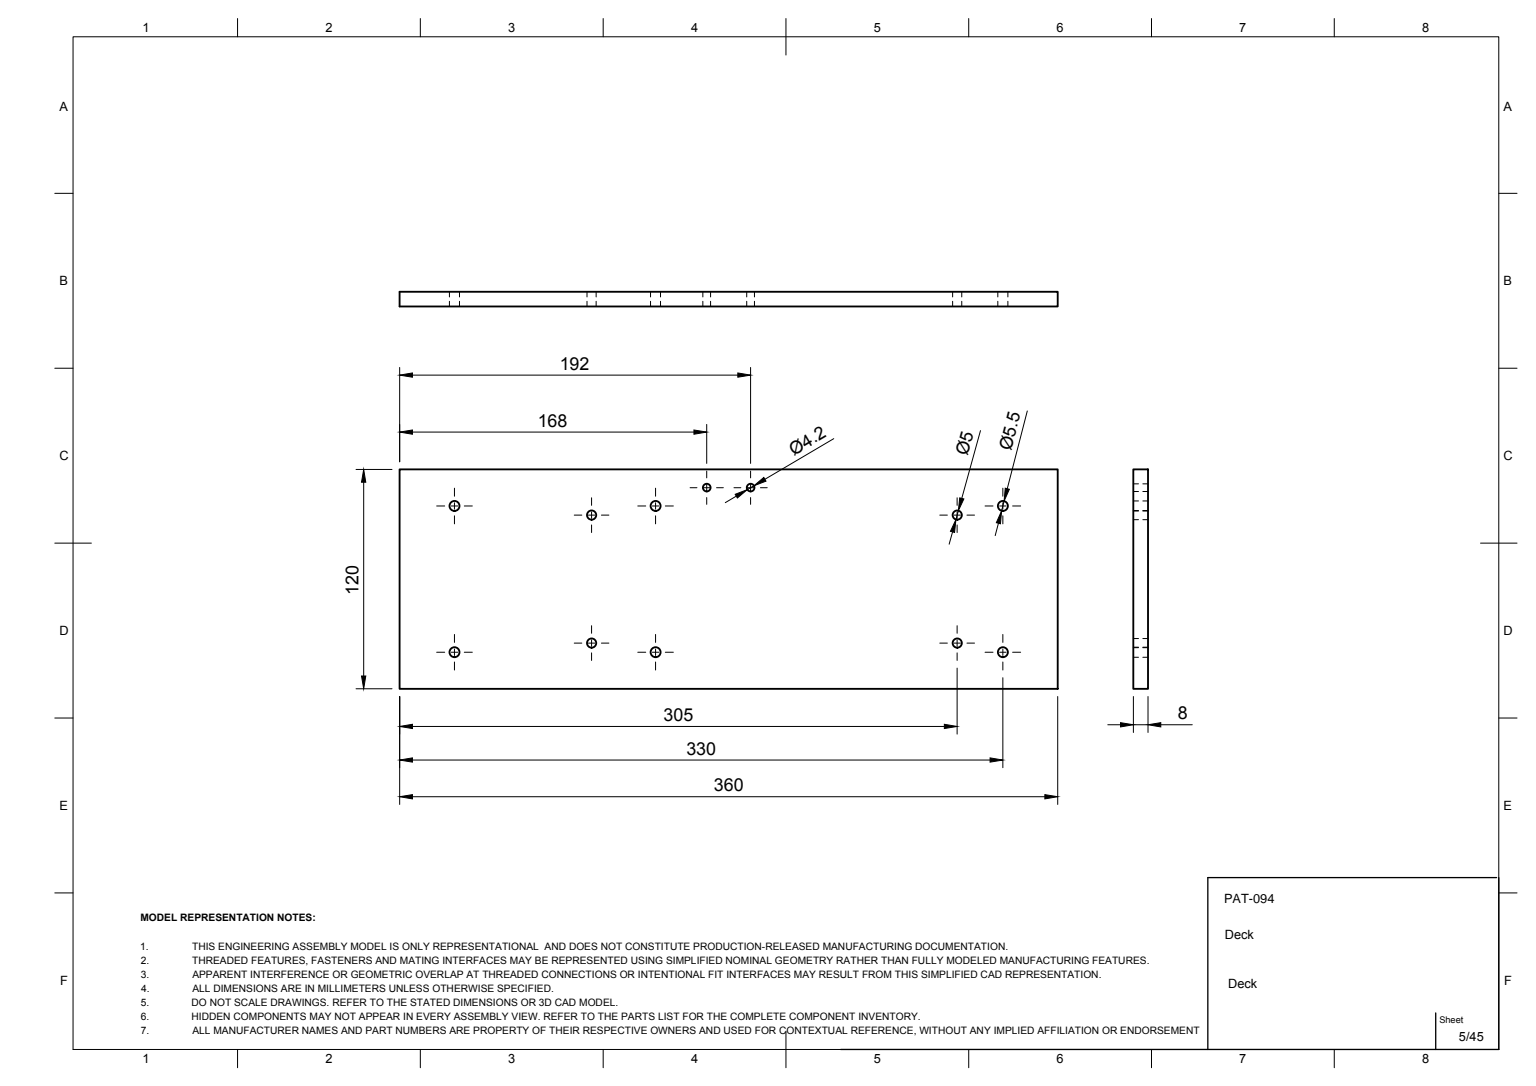
ISO-10303-21;
HEADER;
/* Generated by software containing ST-Developer
 * from STEP Tools, Inc. (www.steptools.com) 
 */

FILE_DESCRIPTION(
/* description */ ('Shaft runout checking stand'),
/* implementation_level */ '2;1');

FILE_NAME(
/* name */ 'Deck.step',
/* time_stamp */ '2026-11-02T21:12:33-08:00',
/* author */ (''),
/* organization */ (''),
/* preprocessor_version */ 'ST-DEVELOPER v20.2',
/* originating_system */ 'Autodesk Translation Framework v15.17.0.0',
/* authorisation */ '');

FILE_SCHEMA (('AUTOMOTIVE_DESIGN { 1 0 10303 214 3 1 1 }'));
ENDSEC;

DATA;
#10=MECHANICAL_DESIGN_GEOMETRIC_PRESENTATION_REPRESENTATION('',(#464),#11748);
#378=SHAPE_REPRESENTATION_RELATIONSHIP('SRR','None',#11927,#421);
#421=ADVANCED_BREP_SHAPE_REPRESENTATION('',(#515),#11703);
#464=STYLED_ITEM('',(#12169),#515);
#515=MANIFOLD_SOLID_BREP('Body1',#6207);
#564=FACE_BOUND('',#1472,.T.);
#565=FACE_BOUND('',#1473,.T.);
#566=FACE_BOUND('',#1474,.T.);
#567=FACE_BOUND('',#1475,.T.);
#568=FACE_BOUND('',#1476,.T.);
#569=FACE_BOUND('',#1477,.T.);
#570=FACE_BOUND('',#1478,.T.);
#571=FACE_BOUND('',#1479,.T.);
#572=FACE_BOUND('',#1480,.T.);
#573=FACE_BOUND('',#1481,.T.);
#574=FACE_BOUND('',#1482,.T.);
#575=FACE_BOUND('',#1483,.T.);
#576=FACE_BOUND('',#1485,.T.);
#577=FACE_BOUND('',#1486,.T.);
#578=FACE_BOUND('',#1487,.T.);
#579=FACE_BOUND('',#1488,.T.);
#580=FACE_BOUND('',#1489,.T.);
#581=FACE_BOUND('',#1490,.T.);
#582=FACE_BOUND('',#1491,.T.);
#583=FACE_BOUND('',#1492,.T.);
#584=FACE_BOUND('',#1493,.T.);
#585=FACE_BOUND('',#1494,.T.);
#586=FACE_BOUND('',#1495,.T.);
#587=FACE_BOUND('',#1496,.T.);
#675=CIRCLE('',#6788,0.21);
#676=CIRCLE('',#6789,0.21);
#677=CIRCLE('',#6791,0.21);
#678=CIRCLE('',#6792,0.21);
#679=CIRCLE('',#6794,0.25);
#680=CIRCLE('',#6795,0.25);
#681=CIRCLE('',#6797,0.25);
#682=CIRCLE('',#6798,0.25);
#683=CIRCLE('',#6800,0.25);
#684=CIRCLE('',#6801,0.25);
#685=CIRCLE('',#6803,0.25);
#686=CIRCLE('',#6804,0.25);
#687=CIRCLE('',#6806,0.275);
#688=CIRCLE('',#6807,0.275);
#689=CIRCLE('',#6809,0.275);
#690=CIRCLE('',#6810,0.275);
#691=CIRCLE('',#6812,0.275);
#692=CIRCLE('',#6813,0.275);
#693=CIRCLE('',#6815,0.275);
#694=CIRCLE('',#6816,0.275);
#695=CIRCLE('',#6818,0.275);
#696=CIRCLE('',#6819,0.275);
#697=CIRCLE('',#6821,0.275);
#698=CIRCLE('',#6822,0.275);
#939=CYLINDRICAL_SURFACE('',#6787,0.21);
#940=CYLINDRICAL_SURFACE('',#6790,0.21);
#941=CYLINDRICAL_SURFACE('',#6793,0.25);
#942=CYLINDRICAL_SURFACE('',#6796,0.25);
#943=CYLINDRICAL_SURFACE('',#6799,0.25);
#944=CYLINDRICAL_SURFACE('',#6802,0.25);
#945=CYLINDRICAL_SURFACE('',#6805,0.275);
#946=CYLINDRICAL_SURFACE('',#6808,0.275);
#947=CYLINDRICAL_SURFACE('',#6811,0.275);
#948=CYLINDRICAL_SURFACE('',#6814,0.275);
#949=CYLINDRICAL_SURFACE('',#6817,0.275);
#950=CYLINDRICAL_SURFACE('',#6820,0.275);
#1085=FACE_OUTER_BOUND('',#1455,.T.);
#1086=FACE_OUTER_BOUND('',#1456,.T.);
#1087=FACE_OUTER_BOUND('',#1457,.T.);
#1088=FACE_OUTER_BOUND('',#1458,.T.);
#1089=FACE_OUTER_BOUND('',#1459,.T.);
#1090=FACE_OUTER_BOUND('',#1460,.T.);
#1091=FACE_OUTER_BOUND('',#1461,.T.);
#1092=FACE_OUTER_BOUND('',#1462,.T.);
#1093=FACE_OUTER_BOUND('',#1463,.T.);
#1094=FACE_OUTER_BOUND('',#1464,.T.);
#1095=FACE_OUTER_BOUND('',#1465,.T.);
#1096=FACE_OUTER_BOUND('',#1466,.T.);
#1097=FACE_OUTER_BOUND('',#1467,.T.);
#1098=FACE_OUTER_BOUND('',#1468,.T.);
#1099=FACE_OUTER_BOUND('',#1469,.T.);
#1100=FACE_OUTER_BOUND('',#1470,.T.);
#1101=FACE_OUTER_BOUND('',#1471,.T.);
#1102=FACE_OUTER_BOUND('',#1484,.T.);
#1455=EDGE_LOOP('',(#4358,#4359,#4360,#4361));
#1456=EDGE_LOOP('',(#4362,#4363,#4364,#4365));
#1457=EDGE_LOOP('',(#4366,#4367,#4368,#4369));
#1458=EDGE_LOOP('',(#4370,#4371,#4372,#4373));
#1459=EDGE_LOOP('',(#4374,#4375,#4376,#4377));
#1460=EDGE_LOOP('',(#4378,#4379,#4380,#4381));
#1461=EDGE_LOOP('',(#4382,#4383,#4384,#4385));
#1462=EDGE_LOOP('',(#4386,#4387,#4388,#4389));
#1463=EDGE_LOOP('',(#4390,#4391,#4392,#4393));
#1464=EDGE_LOOP('',(#4394,#4395,#4396,#4397));
#1465=EDGE_LOOP('',(#4398,#4399,#4400,#4401));
#1466=EDGE_LOOP('',(#4402,#4403,#4404,#4405));
#1467=EDGE_LOOP('',(#4406,#4407,#4408,#4409));
#1468=EDGE_LOOP('',(#4410,#4411,#4412,#4413));
#1469=EDGE_LOOP('',(#4414,#4415,#4416,#4417));
#1470=EDGE_LOOP('',(#4418,#4419,#4420,#4421));
#1471=EDGE_LOOP('',(#4422,#4423,#4424,#4425));
#1472=EDGE_LOOP('',(#4426));
#1473=EDGE_LOOP('',(#4427));
#1474=EDGE_LOOP('',(#4428));
#1475=EDGE_LOOP('',(#4429));
#1476=EDGE_LOOP('',(#4430));
#1477=EDGE_LOOP('',(#4431));
#1478=EDGE_LOOP('',(#4432));
#1479=EDGE_LOOP('',(#4433));
#1480=EDGE_LOOP('',(#4434));
#1481=EDGE_LOOP('',(#4435));
#1482=EDGE_LOOP('',(#4436));
#1483=EDGE_LOOP('',(#4437));
#1484=EDGE_LOOP('',(#4438,#4439,#4440,#4441));
#1485=EDGE_LOOP('',(#4442));
#1486=EDGE_LOOP('',(#4443));
#1487=EDGE_LOOP('',(#4444));
#1488=EDGE_LOOP('',(#4445));
#1489=EDGE_LOOP('',(#4446));
#1490=EDGE_LOOP('',(#4447));
#1491=EDGE_LOOP('',(#4448));
#1492=EDGE_LOOP('',(#4449));
#1493=EDGE_LOOP('',(#4450));
#1494=EDGE_LOOP('',(#4451));
#1495=EDGE_LOOP('',(#4452));
#1496=EDGE_LOOP('',(#4453));
#2018=LINE('',#9755,#2485);
#2019=LINE('',#9761,#2486);
#2020=LINE('',#9767,#2487);
#2021=LINE('',#9773,#2488);
#2022=LINE('',#9779,#2489);
#2023=LINE('',#9785,#2490);
#2024=LINE('',#9791,#2491);
#2025=LINE('',#9797,#2492);
#2026=LINE('',#9803,#2493);
#2027=LINE('',#9809,#2494);
#2028=LINE('',#9815,#2495);
#2029=LINE('',#9821,#2496);
#2030=LINE('',#9826,#2497);
#2031=LINE('',#9828,#2498);
#2032=LINE('',#9830,#2499);
#2033=LINE('',#9831,#2500);
#2034=LINE('',#9834,#2501);
#2035=LINE('',#9836,#2502);
#2036=LINE('',#9837,#2503);
#2037=LINE('',#9840,#2504);
#2038=LINE('',#9842,#2505);
#2039=LINE('',#9843,#2506);
#2040=LINE('',#9845,#2507);
#2041=LINE('',#9846,#2508);
#2485=VECTOR('',#7735,0.21);
#2486=VECTOR('',#7742,0.21);
#2487=VECTOR('',#7749,0.25);
#2488=VECTOR('',#7756,0.25);
#2489=VECTOR('',#7763,0.25);
#2490=VECTOR('',#7770,0.25);
#2491=VECTOR('',#7777,0.275);
#2492=VECTOR('',#7784,0.275);
#2493=VECTOR('',#7791,0.275);
#2494=VECTOR('',#7798,0.275);
#2495=VECTOR('',#7805,0.275);
#2496=VECTOR('',#7812,0.275);
#2497=VECTOR('',#7817,1.);
#2498=VECTOR('',#7818,1.);
#2499=VECTOR('',#7819,1.);
#2500=VECTOR('',#7820,1.);
#2501=VECTOR('',#7823,1.);
#2502=VECTOR('',#7824,1.);
#2503=VECTOR('',#7825,1.);
#2504=VECTOR('',#7828,1.);
#2505=VECTOR('',#7829,1.);
#2506=VECTOR('',#7830,1.);
#2507=VECTOR('',#7833,1.);
#2508=VECTOR('',#7834,1.);
#2909=VERTEX_POINT('',#9752);
#2910=VERTEX_POINT('',#9754);
#2911=VERTEX_POINT('',#9758);
#2912=VERTEX_POINT('',#9760);
#2913=VERTEX_POINT('',#9764);
#2914=VERTEX_POINT('',#9766);
#2915=VERTEX_POINT('',#9770);
#2916=VERTEX_POINT('',#9772);
#2917=VERTEX_POINT('',#9776);
#2918=VERTEX_POINT('',#9778);
#2919=VERTEX_POINT('',#9782);
#2920=VERTEX_POINT('',#9784);
#2921=VERTEX_POINT('',#9788);
#2922=VERTEX_POINT('',#9790);
#2923=VERTEX_POINT('',#9794);
#2924=VERTEX_POINT('',#9796);
#2925=VERTEX_POINT('',#9800);
#2926=VERTEX_POINT('',#9802);
#2927=VERTEX_POINT('',#9806);
#2928=VERTEX_POINT('',#9808);
#2929=VERTEX_POINT('',#9812);
#2930=VERTEX_POINT('',#9814);
#2931=VERTEX_POINT('',#9818);
#2932=VERTEX_POINT('',#9820);
#2933=VERTEX_POINT('',#9824);
#2934=VERTEX_POINT('',#9825);
#2935=VERTEX_POINT('',#9827);
#2936=VERTEX_POINT('',#9829);
#2937=VERTEX_POINT('',#9833);
#2938=VERTEX_POINT('',#9835);
#2939=VERTEX_POINT('',#9839);
#2940=VERTEX_POINT('',#9841);
#3465=EDGE_CURVE('',#2909,#2909,#675,.T.);
#3466=EDGE_CURVE('',#2909,#2910,#2018,.T.);
#3467=EDGE_CURVE('',#2910,#2910,#676,.T.);
#3468=EDGE_CURVE('',#2911,#2911,#677,.T.);
#3469=EDGE_CURVE('',#2911,#2912,#2019,.T.);
#3470=EDGE_CURVE('',#2912,#2912,#678,.T.);
#3471=EDGE_CURVE('',#2913,#2913,#679,.T.);
#3472=EDGE_CURVE('',#2913,#2914,#2020,.T.);
#3473=EDGE_CURVE('',#2914,#2914,#680,.T.);
#3474=EDGE_CURVE('',#2915,#2915,#681,.T.);
#3475=EDGE_CURVE('',#2915,#2916,#2021,.T.);
#3476=EDGE_CURVE('',#2916,#2916,#682,.T.);
#3477=EDGE_CURVE('',#2917,#2917,#683,.T.);
#3478=EDGE_CURVE('',#2917,#2918,#2022,.T.);
#3479=EDGE_CURVE('',#2918,#2918,#684,.T.);
#3480=EDGE_CURVE('',#2919,#2919,#685,.T.);
#3481=EDGE_CURVE('',#2919,#2920,#2023,.T.);
#3482=EDGE_CURVE('',#2920,#2920,#686,.T.);
#3483=EDGE_CURVE('',#2921,#2921,#687,.T.);
#3484=EDGE_CURVE('',#2921,#2922,#2024,.T.);
#3485=EDGE_CURVE('',#2922,#2922,#688,.T.);
#3486=EDGE_CURVE('',#2923,#2923,#689,.T.);
#3487=EDGE_CURVE('',#2923,#2924,#2025,.T.);
#3488=EDGE_CURVE('',#2924,#2924,#690,.T.);
#3489=EDGE_CURVE('',#2925,#2925,#691,.T.);
#3490=EDGE_CURVE('',#2925,#2926,#2026,.T.);
#3491=EDGE_CURVE('',#2926,#2926,#692,.T.);
#3492=EDGE_CURVE('',#2927,#2927,#693,.T.);
#3493=EDGE_CURVE('',#2927,#2928,#2027,.T.);
#3494=EDGE_CURVE('',#2928,#2928,#694,.T.);
#3495=EDGE_CURVE('',#2929,#2929,#695,.T.);
#3496=EDGE_CURVE('',#2929,#2930,#2028,.T.);
#3497=EDGE_CURVE('',#2930,#2930,#696,.T.);
#3498=EDGE_CURVE('',#2931,#2931,#697,.T.);
#3499=EDGE_CURVE('',#2931,#2932,#2029,.T.);
#3500=EDGE_CURVE('',#2932,#2932,#698,.T.);
#3501=EDGE_CURVE('',#2933,#2934,#2030,.T.);
#3502=EDGE_CURVE('',#2934,#2935,#2031,.T.);
#3503=EDGE_CURVE('',#2936,#2935,#2032,.T.);
#3504=EDGE_CURVE('',#2933,#2936,#2033,.T.);
#3505=EDGE_CURVE('',#2937,#2933,#2034,.T.);
#3506=EDGE_CURVE('',#2938,#2936,#2035,.T.);
#3507=EDGE_CURVE('',#2937,#2938,#2036,.T.);
#3508=EDGE_CURVE('',#2939,#2937,#2037,.T.);
#3509=EDGE_CURVE('',#2940,#2938,#2038,.T.);
#3510=EDGE_CURVE('',#2939,#2940,#2039,.T.);
#3511=EDGE_CURVE('',#2934,#2939,#2040,.T.);
#3512=EDGE_CURVE('',#2935,#2940,#2041,.T.);
#4358=ORIENTED_EDGE('',*,*,#3465,.F.);
#4359=ORIENTED_EDGE('',*,*,#3466,.T.);
#4360=ORIENTED_EDGE('',*,*,#3467,.F.);
#4361=ORIENTED_EDGE('',*,*,#3466,.F.);
#4362=ORIENTED_EDGE('',*,*,#3468,.F.);
#4363=ORIENTED_EDGE('',*,*,#3469,.T.);
#4364=ORIENTED_EDGE('',*,*,#3470,.F.);
#4365=ORIENTED_EDGE('',*,*,#3469,.F.);
#4366=ORIENTED_EDGE('',*,*,#3471,.F.);
#4367=ORIENTED_EDGE('',*,*,#3472,.T.);
#4368=ORIENTED_EDGE('',*,*,#3473,.F.);
#4369=ORIENTED_EDGE('',*,*,#3472,.F.);
#4370=ORIENTED_EDGE('',*,*,#3474,.F.);
#4371=ORIENTED_EDGE('',*,*,#3475,.T.);
#4372=ORIENTED_EDGE('',*,*,#3476,.F.);
#4373=ORIENTED_EDGE('',*,*,#3475,.F.);
#4374=ORIENTED_EDGE('',*,*,#3477,.F.);
#4375=ORIENTED_EDGE('',*,*,#3478,.T.);
#4376=ORIENTED_EDGE('',*,*,#3479,.F.);
#4377=ORIENTED_EDGE('',*,*,#3478,.F.);
#4378=ORIENTED_EDGE('',*,*,#3480,.F.);
#4379=ORIENTED_EDGE('',*,*,#3481,.T.);
#4380=ORIENTED_EDGE('',*,*,#3482,.F.);
#4381=ORIENTED_EDGE('',*,*,#3481,.F.);
#4382=ORIENTED_EDGE('',*,*,#3483,.F.);
#4383=ORIENTED_EDGE('',*,*,#3484,.T.);
#4384=ORIENTED_EDGE('',*,*,#3485,.F.);
#4385=ORIENTED_EDGE('',*,*,#3484,.F.);
#4386=ORIENTED_EDGE('',*,*,#3486,.F.);
#4387=ORIENTED_EDGE('',*,*,#3487,.T.);
#4388=ORIENTED_EDGE('',*,*,#3488,.F.);
#4389=ORIENTED_EDGE('',*,*,#3487,.F.);
#4390=ORIENTED_EDGE('',*,*,#3489,.F.);
#4391=ORIENTED_EDGE('',*,*,#3490,.T.);
#4392=ORIENTED_EDGE('',*,*,#3491,.F.);
#4393=ORIENTED_EDGE('',*,*,#3490,.F.);
#4394=ORIENTED_EDGE('',*,*,#3492,.F.);
#4395=ORIENTED_EDGE('',*,*,#3493,.T.);
#4396=ORIENTED_EDGE('',*,*,#3494,.F.);
#4397=ORIENTED_EDGE('',*,*,#3493,.F.);
#4398=ORIENTED_EDGE('',*,*,#3495,.F.);
#4399=ORIENTED_EDGE('',*,*,#3496,.T.);
#4400=ORIENTED_EDGE('',*,*,#3497,.F.);
#4401=ORIENTED_EDGE('',*,*,#3496,.F.);
#4402=ORIENTED_EDGE('',*,*,#3498,.F.);
#4403=ORIENTED_EDGE('',*,*,#3499,.T.);
#4404=ORIENTED_EDGE('',*,*,#3500,.F.);
#4405=ORIENTED_EDGE('',*,*,#3499,.F.);
#4406=ORIENTED_EDGE('',*,*,#3501,.T.);
#4407=ORIENTED_EDGE('',*,*,#3502,.T.);
#4408=ORIENTED_EDGE('',*,*,#3503,.F.);
#4409=ORIENTED_EDGE('',*,*,#3504,.F.);
#4410=ORIENTED_EDGE('',*,*,#3505,.T.);
#4411=ORIENTED_EDGE('',*,*,#3504,.T.);
#4412=ORIENTED_EDGE('',*,*,#3506,.F.);
#4413=ORIENTED_EDGE('',*,*,#3507,.F.);
#4414=ORIENTED_EDGE('',*,*,#3508,.T.);
#4415=ORIENTED_EDGE('',*,*,#3507,.T.);
#4416=ORIENTED_EDGE('',*,*,#3509,.F.);
#4417=ORIENTED_EDGE('',*,*,#3510,.F.);
#4418=ORIENTED_EDGE('',*,*,#3511,.T.);
#4419=ORIENTED_EDGE('',*,*,#3510,.T.);
#4420=ORIENTED_EDGE('',*,*,#3512,.F.);
#4421=ORIENTED_EDGE('',*,*,#3502,.F.);
#4422=ORIENTED_EDGE('',*,*,#3512,.T.);
#4423=ORIENTED_EDGE('',*,*,#3509,.T.);
#4424=ORIENTED_EDGE('',*,*,#3506,.T.);
#4425=ORIENTED_EDGE('',*,*,#3503,.T.);
#4426=ORIENTED_EDGE('',*,*,#3473,.T.);
#4427=ORIENTED_EDGE('',*,*,#3476,.T.);
#4428=ORIENTED_EDGE('',*,*,#3485,.T.);
#4429=ORIENTED_EDGE('',*,*,#3488,.T.);
#4430=ORIENTED_EDGE('',*,*,#3491,.T.);
#4431=ORIENTED_EDGE('',*,*,#3494,.T.);
#4432=ORIENTED_EDGE('',*,*,#3497,.T.);
#4433=ORIENTED_EDGE('',*,*,#3500,.T.);
#4434=ORIENTED_EDGE('',*,*,#3482,.T.);
#4435=ORIENTED_EDGE('',*,*,#3479,.T.);
#4436=ORIENTED_EDGE('',*,*,#3470,.T.);
#4437=ORIENTED_EDGE('',*,*,#3467,.T.);
#4438=ORIENTED_EDGE('',*,*,#3511,.F.);
#4439=ORIENTED_EDGE('',*,*,#3501,.F.);
#4440=ORIENTED_EDGE('',*,*,#3505,.F.);
#4441=ORIENTED_EDGE('',*,*,#3508,.F.);
#4442=ORIENTED_EDGE('',*,*,#3471,.T.);
#4443=ORIENTED_EDGE('',*,*,#3474,.T.);
#4444=ORIENTED_EDGE('',*,*,#3483,.T.);
#4445=ORIENTED_EDGE('',*,*,#3486,.T.);
#4446=ORIENTED_EDGE('',*,*,#3489,.T.);
#4447=ORIENTED_EDGE('',*,*,#3492,.T.);
#4448=ORIENTED_EDGE('',*,*,#3495,.T.);
#4449=ORIENTED_EDGE('',*,*,#3498,.T.);
#4450=ORIENTED_EDGE('',*,*,#3480,.T.);
#4451=ORIENTED_EDGE('',*,*,#3477,.T.);
#4452=ORIENTED_EDGE('',*,*,#3468,.T.);
#4453=ORIENTED_EDGE('',*,*,#3465,.T.);
#5650=PLANE('',#6823);
#5651=PLANE('',#6824);
#5652=PLANE('',#6825);
#5653=PLANE('',#6826);
#5654=PLANE('',#6827);
#5655=PLANE('',#6828);
#5885=ADVANCED_FACE('',(#1085),#939,.F.);
#5886=ADVANCED_FACE('',(#1086),#940,.F.);
#5887=ADVANCED_FACE('',(#1087),#941,.F.);
#5888=ADVANCED_FACE('',(#1088),#942,.F.);
#5889=ADVANCED_FACE('',(#1089),#943,.F.);
#5890=ADVANCED_FACE('',(#1090),#944,.F.);
#5891=ADVANCED_FACE('',(#1091),#945,.F.);
#5892=ADVANCED_FACE('',(#1092),#946,.F.);
#5893=ADVANCED_FACE('',(#1093),#947,.F.);
#5894=ADVANCED_FACE('',(#1094),#948,.F.);
#5895=ADVANCED_FACE('',(#1095),#949,.F.);
#5896=ADVANCED_FACE('',(#1096),#950,.F.);
#5897=ADVANCED_FACE('',(#1097),#5650,.T.);
#5898=ADVANCED_FACE('',(#1098),#5651,.T.);
#5899=ADVANCED_FACE('',(#1099),#5652,.T.);
#5900=ADVANCED_FACE('',(#1100),#5653,.T.);
#5901=ADVANCED_FACE('',(#1101,#564,#565,#566,#567,#568,#569,#570,#571,#572,
#573,#574,#575),#5654,.T.);
#5902=ADVANCED_FACE('',(#1102,#576,#577,#578,#579,#580,#581,#582,#583,#584,
#585,#586,#587),#5655,.F.);
#6207=CLOSED_SHELL('',(#5885,#5886,#5887,#5888,#5889,#5890,#5891,#5892,
#5893,#5894,#5895,#5896,#5897,#5898,#5899,#5900,#5901,#5902));
#6786=AXIS2_PLACEMENT_3D('',#9750,#7729,#7730);
#6787=AXIS2_PLACEMENT_3D('',#9751,#7731,#7732);
#6788=AXIS2_PLACEMENT_3D('',#9753,#7733,#7734);
#6789=AXIS2_PLACEMENT_3D('',#9756,#7736,#7737);
#6790=AXIS2_PLACEMENT_3D('',#9757,#7738,#7739);
#6791=AXIS2_PLACEMENT_3D('',#9759,#7740,#7741);
#6792=AXIS2_PLACEMENT_3D('',#9762,#7743,#7744);
#6793=AXIS2_PLACEMENT_3D('',#9763,#7745,#7746);
#6794=AXIS2_PLACEMENT_3D('',#9765,#7747,#7748);
#6795=AXIS2_PLACEMENT_3D('',#9768,#7750,#7751);
#6796=AXIS2_PLACEMENT_3D('',#9769,#7752,#7753);
#6797=AXIS2_PLACEMENT_3D('',#9771,#7754,#7755);
#6798=AXIS2_PLACEMENT_3D('',#9774,#7757,#7758);
#6799=AXIS2_PLACEMENT_3D('',#9775,#7759,#7760);
#6800=AXIS2_PLACEMENT_3D('',#9777,#7761,#7762);
#6801=AXIS2_PLACEMENT_3D('',#9780,#7764,#7765);
#6802=AXIS2_PLACEMENT_3D('',#9781,#7766,#7767);
#6803=AXIS2_PLACEMENT_3D('',#9783,#7768,#7769);
#6804=AXIS2_PLACEMENT_3D('',#9786,#7771,#7772);
#6805=AXIS2_PLACEMENT_3D('',#9787,#7773,#7774);
#6806=AXIS2_PLACEMENT_3D('',#9789,#7775,#7776);
#6807=AXIS2_PLACEMENT_3D('',#9792,#7778,#7779);
#6808=AXIS2_PLACEMENT_3D('',#9793,#7780,#7781);
#6809=AXIS2_PLACEMENT_3D('',#9795,#7782,#7783);
#6810=AXIS2_PLACEMENT_3D('',#9798,#7785,#7786);
#6811=AXIS2_PLACEMENT_3D('',#9799,#7787,#7788);
#6812=AXIS2_PLACEMENT_3D('',#9801,#7789,#7790);
#6813=AXIS2_PLACEMENT_3D('',#9804,#7792,#7793);
#6814=AXIS2_PLACEMENT_3D('',#9805,#7794,#7795);
#6815=AXIS2_PLACEMENT_3D('',#9807,#7796,#7797);
#6816=AXIS2_PLACEMENT_3D('',#9810,#7799,#7800);
#6817=AXIS2_PLACEMENT_3D('',#9811,#7801,#7802);
#6818=AXIS2_PLACEMENT_3D('',#9813,#7803,#7804);
#6819=AXIS2_PLACEMENT_3D('',#9816,#7806,#7807);
#6820=AXIS2_PLACEMENT_3D('',#9817,#7808,#7809);
#6821=AXIS2_PLACEMENT_3D('',#9819,#7810,#7811);
#6822=AXIS2_PLACEMENT_3D('',#9822,#7813,#7814);
#6823=AXIS2_PLACEMENT_3D('',#9823,#7815,#7816);
#6824=AXIS2_PLACEMENT_3D('',#9832,#7821,#7822);
#6825=AXIS2_PLACEMENT_3D('',#9838,#7826,#7827);
#6826=AXIS2_PLACEMENT_3D('',#9844,#7831,#7832);
#6827=AXIS2_PLACEMENT_3D('',#9847,#7835,#7836);
#6828=AXIS2_PLACEMENT_3D('',#9848,#7837,#7838);
#7729=DIRECTION('axis',(0.,0.,1.));
#7730=DIRECTION('refdir',(1.,0.,0.));
#7731=DIRECTION('center_axis',(0.,0.,1.));
#7732=DIRECTION('ref_axis',(1.,0.,0.));
#7733=DIRECTION('center_axis',(0.,0.,1.));
#7734=DIRECTION('ref_axis',(1.,0.,0.));
#7735=DIRECTION('',(0.,0.,1.));
#7736=DIRECTION('center_axis',(0.,0.,-1.));
#7737=DIRECTION('ref_axis',(1.,0.,0.));
#7738=DIRECTION('center_axis',(0.,0.,1.));
#7739=DIRECTION('ref_axis',(1.,0.,0.));
#7740=DIRECTION('center_axis',(0.,0.,1.));
#7741=DIRECTION('ref_axis',(1.,0.,0.));
#7742=DIRECTION('',(0.,0.,1.));
#7743=DIRECTION('center_axis',(0.,0.,-1.));
#7744=DIRECTION('ref_axis',(1.,0.,0.));
#7745=DIRECTION('center_axis',(0.,0.,1.));
#7746=DIRECTION('ref_axis',(1.,0.,0.));
#7747=DIRECTION('center_axis',(0.,0.,1.));
#7748=DIRECTION('ref_axis',(1.,0.,0.));
#7749=DIRECTION('',(0.,0.,1.));
#7750=DIRECTION('center_axis',(0.,0.,-1.));
#7751=DIRECTION('ref_axis',(1.,0.,0.));
#7752=DIRECTION('center_axis',(0.,0.,1.));
#7753=DIRECTION('ref_axis',(1.,0.,0.));
#7754=DIRECTION('center_axis',(0.,0.,1.));
#7755=DIRECTION('ref_axis',(1.,0.,0.));
#7756=DIRECTION('',(0.,0.,1.));
#7757=DIRECTION('center_axis',(0.,0.,-1.));
#7758=DIRECTION('ref_axis',(1.,0.,0.));
#7759=DIRECTION('center_axis',(0.,0.,1.));
#7760=DIRECTION('ref_axis',(1.,0.,0.));
#7761=DIRECTION('center_axis',(0.,0.,1.));
#7762=DIRECTION('ref_axis',(1.,0.,0.));
#7763=DIRECTION('',(0.,0.,1.));
#7764=DIRECTION('center_axis',(0.,0.,-1.));
#7765=DIRECTION('ref_axis',(1.,0.,0.));
#7766=DIRECTION('center_axis',(0.,0.,1.));
#7767=DIRECTION('ref_axis',(1.,0.,0.));
#7768=DIRECTION('center_axis',(0.,0.,1.));
#7769=DIRECTION('ref_axis',(1.,0.,0.));
#7770=DIRECTION('',(0.,0.,1.));
#7771=DIRECTION('center_axis',(0.,0.,-1.));
#7772=DIRECTION('ref_axis',(1.,0.,0.));
#7773=DIRECTION('center_axis',(0.,0.,1.));
#7774=DIRECTION('ref_axis',(1.,0.,0.));
#7775=DIRECTION('center_axis',(0.,0.,1.));
#7776=DIRECTION('ref_axis',(1.,0.,0.));
#7777=DIRECTION('',(0.,0.,1.));
#7778=DIRECTION('center_axis',(0.,0.,-1.));
#7779=DIRECTION('ref_axis',(1.,0.,0.));
#7780=DIRECTION('center_axis',(0.,0.,1.));
#7781=DIRECTION('ref_axis',(1.,0.,0.));
#7782=DIRECTION('center_axis',(0.,0.,1.));
#7783=DIRECTION('ref_axis',(1.,0.,0.));
#7784=DIRECTION('',(0.,0.,1.));
#7785=DIRECTION('center_axis',(0.,0.,-1.));
#7786=DIRECTION('ref_axis',(1.,0.,0.));
#7787=DIRECTION('center_axis',(0.,0.,1.));
#7788=DIRECTION('ref_axis',(1.,0.,0.));
#7789=DIRECTION('center_axis',(0.,0.,1.));
#7790=DIRECTION('ref_axis',(1.,0.,0.));
#7791=DIRECTION('',(0.,0.,1.));
#7792=DIRECTION('center_axis',(0.,0.,-1.));
#7793=DIRECTION('ref_axis',(1.,0.,0.));
#7794=DIRECTION('center_axis',(0.,0.,1.));
#7795=DIRECTION('ref_axis',(1.,0.,0.));
#7796=DIRECTION('center_axis',(0.,0.,1.));
#7797=DIRECTION('ref_axis',(1.,0.,0.));
#7798=DIRECTION('',(0.,0.,1.));
#7799=DIRECTION('center_axis',(0.,0.,-1.));
#7800=DIRECTION('ref_axis',(1.,0.,0.));
#7801=DIRECTION('center_axis',(0.,0.,1.));
#7802=DIRECTION('ref_axis',(1.,0.,0.));
#7803=DIRECTION('center_axis',(0.,0.,1.));
#7804=DIRECTION('ref_axis',(1.,0.,0.));
#7805=DIRECTION('',(0.,0.,1.));
#7806=DIRECTION('center_axis',(0.,0.,-1.));
#7807=DIRECTION('ref_axis',(1.,0.,0.));
#7808=DIRECTION('center_axis',(0.,0.,1.));
#7809=DIRECTION('ref_axis',(1.,0.,0.));
#7810=DIRECTION('center_axis',(0.,0.,1.));
#7811=DIRECTION('ref_axis',(1.,0.,0.));
#7812=DIRECTION('',(0.,0.,1.));
#7813=DIRECTION('center_axis',(0.,0.,-1.));
#7814=DIRECTION('ref_axis',(1.,0.,0.));
#7815=DIRECTION('center_axis',(0.,1.,0.));
#7816=DIRECTION('ref_axis',(-1.,0.,0.));
#7817=DIRECTION('',(-1.,0.,0.));
#7818=DIRECTION('',(0.,0.,1.));
#7819=DIRECTION('',(-1.,0.,0.));
#7820=DIRECTION('',(0.,0.,1.));
#7821=DIRECTION('center_axis',(1.,0.,0.));
#7822=DIRECTION('ref_axis',(0.,1.,0.));
#7823=DIRECTION('',(0.,1.,0.));
#7824=DIRECTION('',(0.,1.,0.));
#7825=DIRECTION('',(0.,0.,1.));
#7826=DIRECTION('center_axis',(0.,-1.,0.));
#7827=DIRECTION('ref_axis',(1.,0.,0.));
#7828=DIRECTION('',(1.,0.,0.));
#7829=DIRECTION('',(1.,0.,0.));
#7830=DIRECTION('',(0.,0.,1.));
#7831=DIRECTION('center_axis',(-1.,0.,0.));
#7832=DIRECTION('ref_axis',(0.,-1.,0.));
#7833=DIRECTION('',(0.,-1.,0.));
#7834=DIRECTION('',(0.,-1.,0.));
#7835=DIRECTION('center_axis',(0.,0.,1.));
#7836=DIRECTION('ref_axis',(1.,0.,0.));
#7837=DIRECTION('center_axis',(0.,0.,1.));
#7838=DIRECTION('ref_axis',(1.,0.,0.));
#9750=CARTESIAN_POINT('',(0.,0.,0.));
#9751=CARTESIAN_POINT('Origin',(5.,-1.2,1.9));
#9752=CARTESIAN_POINT('',(4.79,-1.2,2.));
#9753=CARTESIAN_POINT('Origin',(5.,-1.2,2.));
#9754=CARTESIAN_POINT('',(4.79,-1.2,2.8));
#9755=CARTESIAN_POINT('',(4.79,-1.2,1.9));
#9756=CARTESIAN_POINT('Origin',(5.,-1.2,2.8));
#9757=CARTESIAN_POINT('Origin',(5.,1.2,1.9));
#9758=CARTESIAN_POINT('',(4.79,1.2,2.));
#9759=CARTESIAN_POINT('Origin',(5.,1.2,2.));
#9760=CARTESIAN_POINT('',(4.79,1.2,2.8));
#9761=CARTESIAN_POINT('',(4.79,1.2,1.9));
#9762=CARTESIAN_POINT('Origin',(5.,1.2,2.8));
#9763=CARTESIAN_POINT('Origin',(-3.5,7.5,1.9));
#9764=CARTESIAN_POINT('',(-3.75,7.5,2.));
#9765=CARTESIAN_POINT('Origin',(-3.5,7.5,2.));
#9766=CARTESIAN_POINT('',(-3.75,7.5,2.8));
#9767=CARTESIAN_POINT('',(-3.75,7.5,1.9));
#9768=CARTESIAN_POINT('Origin',(-3.5,7.5,2.8));
#9769=CARTESIAN_POINT('Origin',(3.5,7.5,1.9));
#9770=CARTESIAN_POINT('',(3.25,7.5,2.));
#9771=CARTESIAN_POINT('Origin',(3.5,7.5,2.));
#9772=CARTESIAN_POINT('',(3.25,7.5,2.8));
#9773=CARTESIAN_POINT('',(3.25,7.5,1.9));
#9774=CARTESIAN_POINT('Origin',(3.5,7.5,2.8));
#9775=CARTESIAN_POINT('Origin',(-3.5,-12.5,1.9));
#9776=CARTESIAN_POINT('',(-3.75,-12.5,2.));
#9777=CARTESIAN_POINT('Origin',(-3.5,-12.5,2.));
#9778=CARTESIAN_POINT('',(-3.75,-12.5,2.8));
#9779=CARTESIAN_POINT('',(-3.75,-12.5,1.9));
#9780=CARTESIAN_POINT('Origin',(-3.5,-12.5,2.8));
#9781=CARTESIAN_POINT('Origin',(3.5,-12.5,1.9));
#9782=CARTESIAN_POINT('',(3.25,-12.5,2.));
#9783=CARTESIAN_POINT('Origin',(3.5,-12.5,2.));
#9784=CARTESIAN_POINT('',(3.25,-12.5,2.8));
#9785=CARTESIAN_POINT('',(3.25,-12.5,1.9));
#9786=CARTESIAN_POINT('Origin',(3.5,-12.5,2.8));
#9787=CARTESIAN_POINT('Origin',(4.,4.,1.9));
#9788=CARTESIAN_POINT('',(3.725,4.,2.));
#9789=CARTESIAN_POINT('Origin',(4.,4.,2.));
#9790=CARTESIAN_POINT('',(3.725,4.,2.8));
#9791=CARTESIAN_POINT('',(3.725,4.,1.9));
#9792=CARTESIAN_POINT('Origin',(4.,4.,2.8));
#9793=CARTESIAN_POINT('Origin',(-4.,-15.,1.9));
#9794=CARTESIAN_POINT('',(-4.275,-15.,2.));
#9795=CARTESIAN_POINT('Origin',(-4.,-15.,2.));
#9796=CARTESIAN_POINT('',(-4.275,-15.,2.8));
#9797=CARTESIAN_POINT('',(-4.275,-15.,1.9));
#9798=CARTESIAN_POINT('Origin',(-4.,-15.,2.8));
#9799=CARTESIAN_POINT('Origin',(-4.,4.,1.9));
#9800=CARTESIAN_POINT('',(-4.275,4.,2.));
#9801=CARTESIAN_POINT('Origin',(-4.,4.,2.));
#9802=CARTESIAN_POINT('',(-4.275,4.,2.8));
#9803=CARTESIAN_POINT('',(-4.275,4.,1.9));
#9804=CARTESIAN_POINT('Origin',(-4.,4.,2.8));
#9805=CARTESIAN_POINT('Origin',(-4.,15.,1.9));
#9806=CARTESIAN_POINT('',(-4.275,15.,2.));
#9807=CARTESIAN_POINT('Origin',(-4.,15.,2.));
#9808=CARTESIAN_POINT('',(-4.275,15.,2.8));
#9809=CARTESIAN_POINT('',(-4.275,15.,1.9));
#9810=CARTESIAN_POINT('Origin',(-4.,15.,2.8));
#9811=CARTESIAN_POINT('Origin',(4.,-15.,1.9));
#9812=CARTESIAN_POINT('',(3.725,-15.,2.));
#9813=CARTESIAN_POINT('Origin',(4.,-15.,2.));
#9814=CARTESIAN_POINT('',(3.725,-15.,2.8));
#9815=CARTESIAN_POINT('',(3.725,-15.,1.9));
#9816=CARTESIAN_POINT('Origin',(4.,-15.,2.8));
#9817=CARTESIAN_POINT('Origin',(4.,15.,1.9));
#9818=CARTESIAN_POINT('',(3.725,15.,2.));
#9819=CARTESIAN_POINT('Origin',(4.,15.,2.));
#9820=CARTESIAN_POINT('',(3.725,15.,2.8));
#9821=CARTESIAN_POINT('',(3.725,15.,1.9));
#9822=CARTESIAN_POINT('Origin',(4.,15.,2.8));
#9823=CARTESIAN_POINT('Origin',(6.,18.,2.));
#9824=CARTESIAN_POINT('',(6.,18.,2.));
#9825=CARTESIAN_POINT('',(-6.,18.,2.));
#9826=CARTESIAN_POINT('',(6.,18.,2.));
#9827=CARTESIAN_POINT('',(-6.,18.,2.8));
#9828=CARTESIAN_POINT('',(-6.,18.,2.));
#9829=CARTESIAN_POINT('',(6.,18.,2.8));
#9830=CARTESIAN_POINT('',(6.,18.,2.8));
#9831=CARTESIAN_POINT('',(6.,18.,2.));
#9832=CARTESIAN_POINT('Origin',(6.,-18.,2.));
#9833=CARTESIAN_POINT('',(6.,-18.,2.));
#9834=CARTESIAN_POINT('',(6.,-18.,2.));
#9835=CARTESIAN_POINT('',(6.,-18.,2.8));
#9836=CARTESIAN_POINT('',(6.,-18.,2.8));
#9837=CARTESIAN_POINT('',(6.,-18.,2.));
#9838=CARTESIAN_POINT('Origin',(-6.,-18.,2.));
#9839=CARTESIAN_POINT('',(-6.,-18.,2.));
#9840=CARTESIAN_POINT('',(-6.,-18.,2.));
#9841=CARTESIAN_POINT('',(-6.,-18.,2.8));
#9842=CARTESIAN_POINT('',(-6.,-18.,2.8));
#9843=CARTESIAN_POINT('',(-6.,-18.,2.));
#9844=CARTESIAN_POINT('Origin',(-6.,18.,2.));
#9845=CARTESIAN_POINT('',(-6.,18.,2.));
#9846=CARTESIAN_POINT('',(-6.,18.,2.8));
#9847=CARTESIAN_POINT('Origin',(0.,0.,2.8));
#9848=CARTESIAN_POINT('Origin',(0.,0.,2.));
#11654=UNCERTAINTY_MEASURE_WITH_UNIT(LENGTH_MEASURE(0.001),#11749,
'DISTANCE_ACCURACY_VALUE',
'Maximum model space distance between geometric entities at asserted c
onnectivities');
#11699=UNCERTAINTY_MEASURE_WITH_UNIT(LENGTH_MEASURE(0.001),#11749,
'DISTANCE_ACCURACY_VALUE',
'Maximum model space distance between geometric entities at asserted c
onnectivities');
#11703=(
GEOMETRIC_REPRESENTATION_CONTEXT(3)
GLOBAL_UNCERTAINTY_ASSIGNED_CONTEXT((#11654))
GLOBAL_UNIT_ASSIGNED_CONTEXT((#11749,#11751,#11752))
REPRESENTATION_CONTEXT('','3D')
);
#11748=(
GEOMETRIC_REPRESENTATION_CONTEXT(3)
GLOBAL_UNCERTAINTY_ASSIGNED_CONTEXT((#11699))
GLOBAL_UNIT_ASSIGNED_CONTEXT((#11749,#11751,#11752))
REPRESENTATION_CONTEXT('','3D')
);
#11749=(
LENGTH_UNIT()
NAMED_UNIT(*)
SI_UNIT(.CENTI.,.METRE.)
);
#11751=(
NAMED_UNIT(*)
PLANE_ANGLE_UNIT()
SI_UNIT($,.RADIAN.)
);
#11752=(
NAMED_UNIT(*)
SI_UNIT($,.STERADIAN.)
SOLID_ANGLE_UNIT()
);
#11756=SHAPE_DEFINITION_REPRESENTATION(#11804,#11927);
#11804=PRODUCT_DEFINITION_SHAPE('',$,#11976);
#11927=SHAPE_REPRESENTATION('',(#6786),#11703);
#11972=PRODUCT_DEFINITION_CONTEXT('part definition',#12118,'design');
#11976=PRODUCT_DEFINITION('Deck','Deck',#12024,#11972);
#12024=PRODUCT_DEFINITION_FORMATION('',$,#12123);
#12118=APPLICATION_CONTEXT(
'Core Data for Automotive Mechanical Design Process');
#12119=PRODUCT_CONTEXT('part definition',#12118,'mechanical');
#12123=PRODUCT('Deck','Deck','Deck',(#12119));
#12169=PRESENTATION_STYLE_ASSIGNMENT((#12174));
#12174=SURFACE_STYLE_USAGE(.BOTH.,#12179);
#12179=SURFACE_SIDE_STYLE('',(#12184));
#12184=SURFACE_STYLE_FILL_AREA(#12189);
#12189=FILL_AREA_STYLE('CAD Library Painted - Engineering blue',(#12194));
#12194=FILL_AREA_STYLE_COLOUR('CAD Library Painted - Engineering blue',
#12199);
#12199=COLOUR_RGB('CAD Library Painted - Engineering blue',0.12156862745098,
0.356862745098039,0.6);
ENDSEC;
END-ISO-10303-21;
